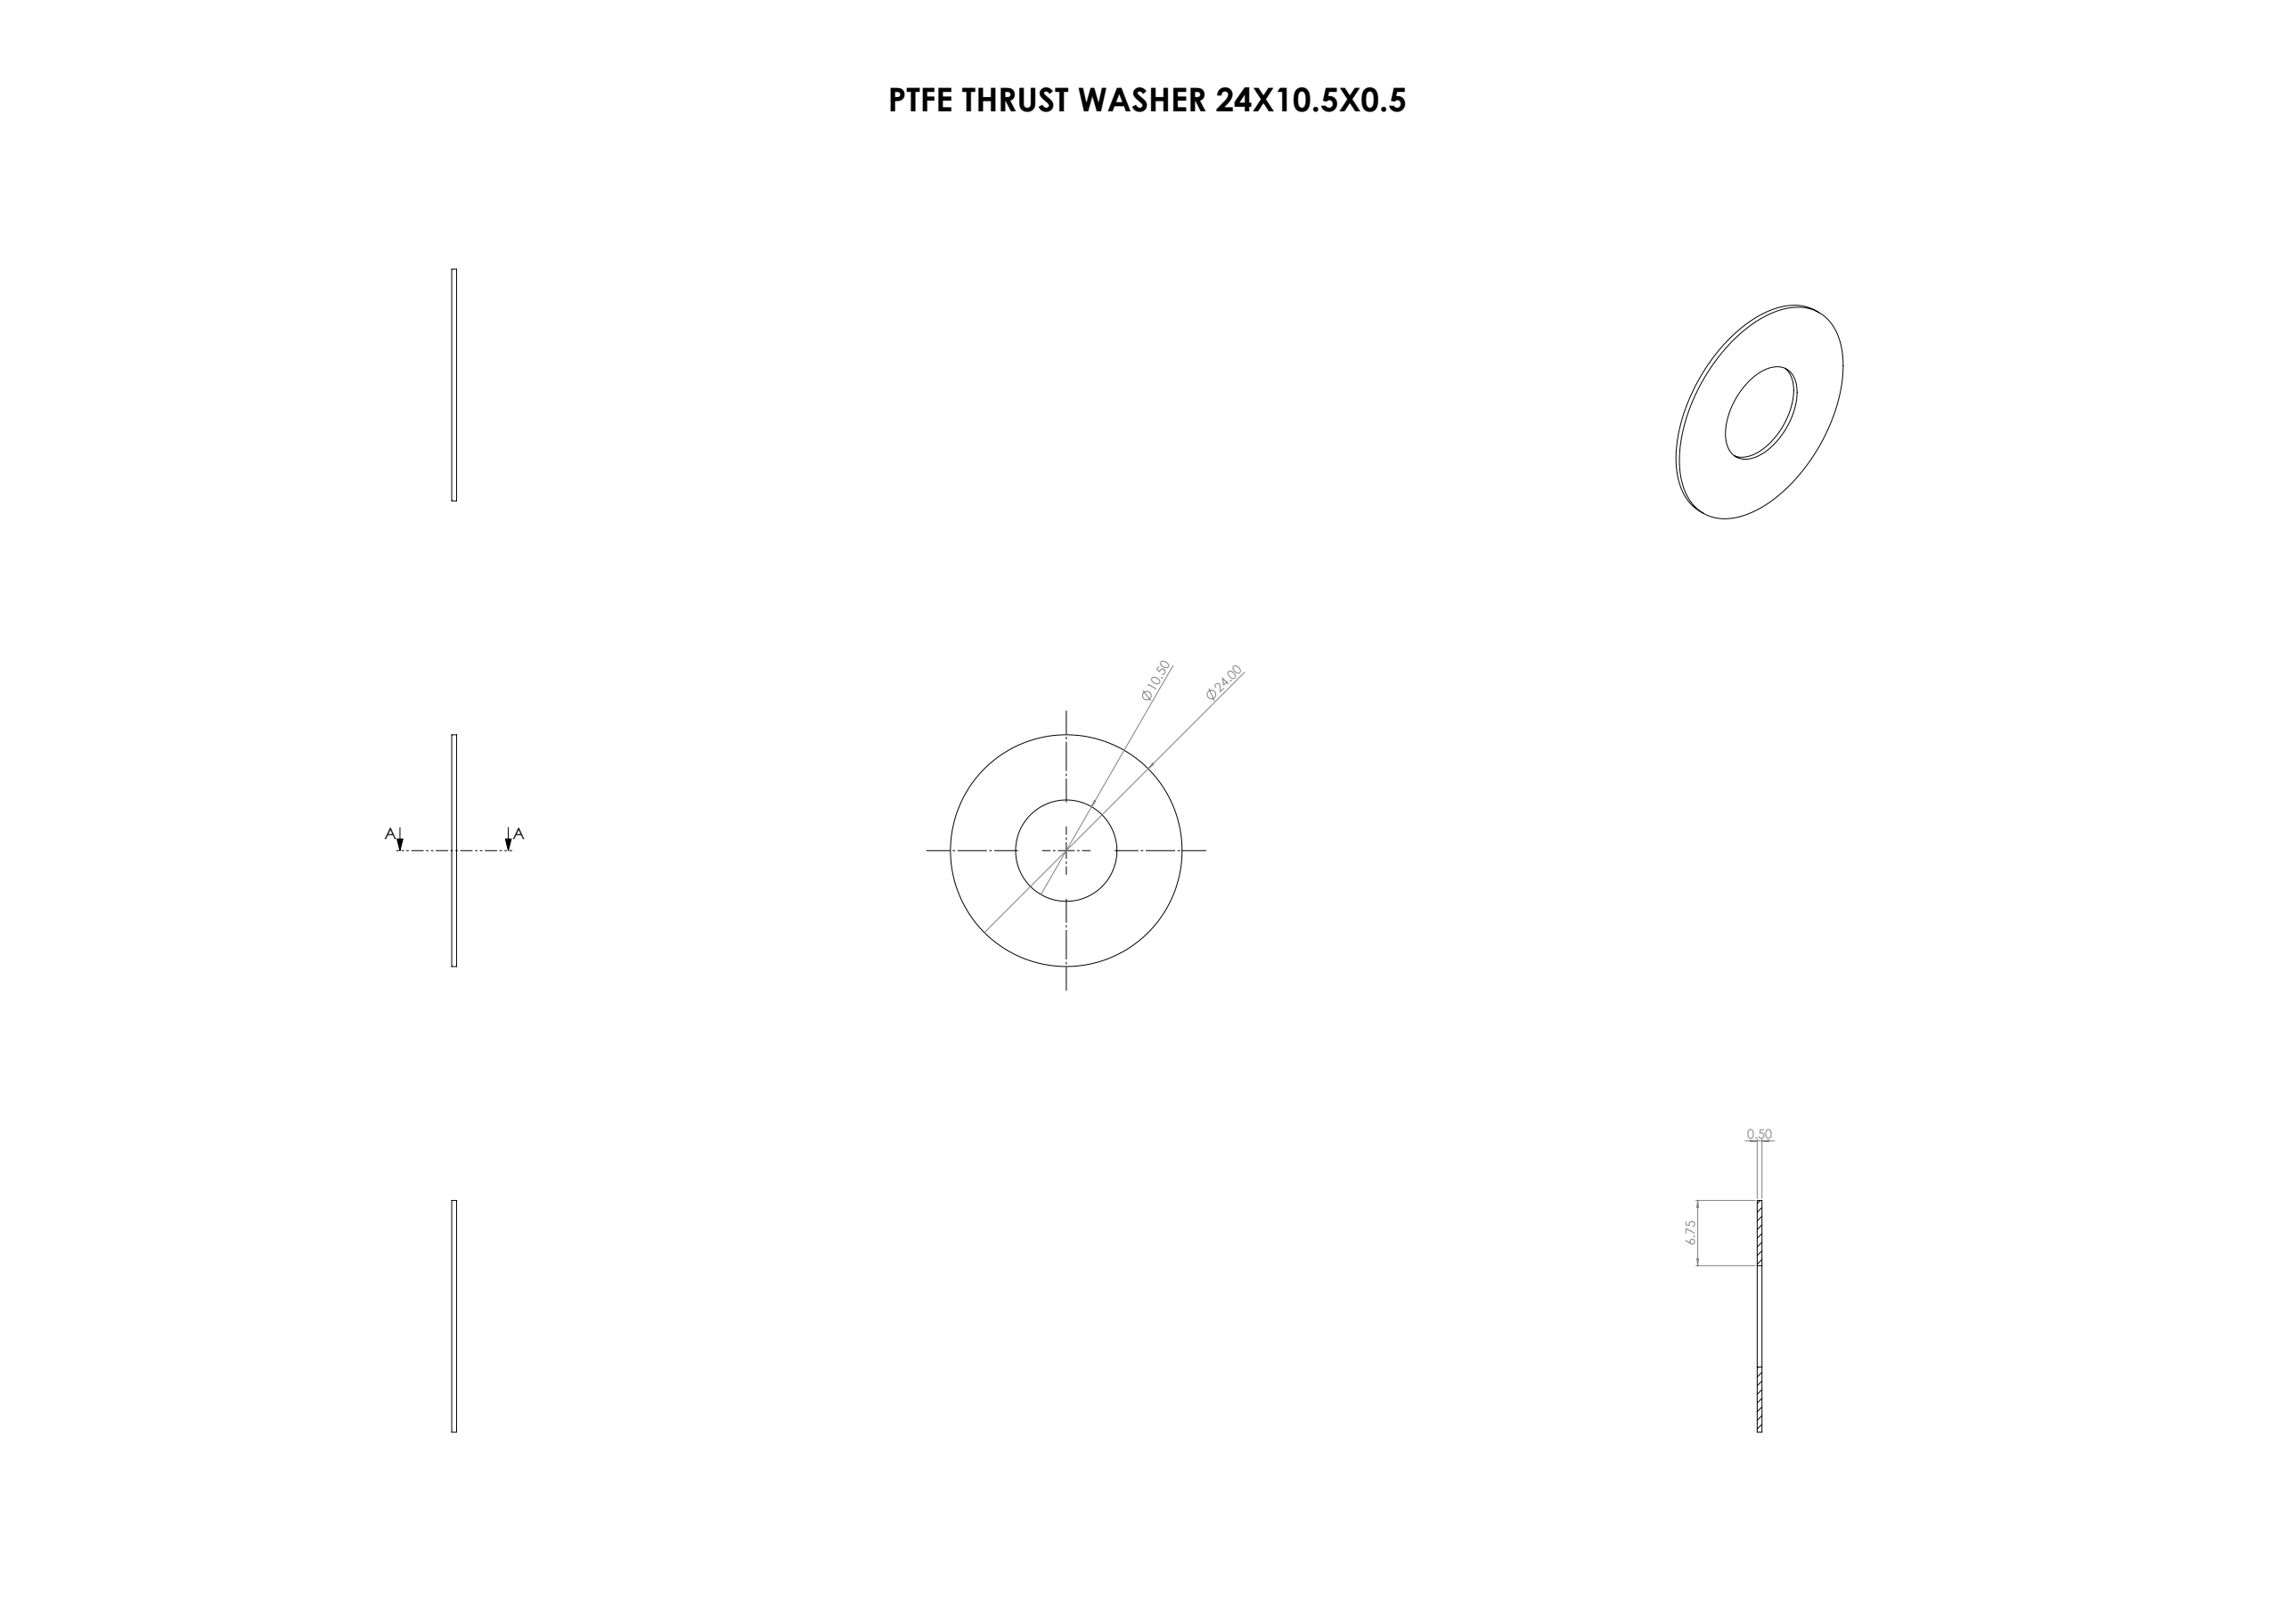
ISO-10303-21;
HEADER;
/* Generated by software containing ST-Developer
 * from STEP Tools, Inc. (www.steptools.com) 
 */

FILE_DESCRIPTION(
/* description */ (''),
/* implementation_level */ '2;1');

FILE_NAME(
/* name */ '06_PTFE_Thrust_Washer_24x10.5x0.5.step',
/* time_stamp */ '2026-10-21T02:03:06-07:00',
/* author */ (''),
/* organization */ (''),
/* preprocessor_version */ 'ST-DEVELOPER v20.2',
/* originating_system */ 'Autodesk Translation Framework v15.15.0.0',
/* authorisation */ '');

FILE_SCHEMA (('AUTOMOTIVE_DESIGN { 1 0 10303 214 3 1 1 }'));
ENDSEC;

DATA;
#10=MECHANICAL_DESIGN_GEOMETRIC_PRESENTATION_REPRESENTATION('',(#120),#38528);
#96=SHAPE_REPRESENTATION_RELATIONSHIP('SRR','None',#38581,#108);
#108=ADVANCED_BREP_SHAPE_REPRESENTATION('',(#132),#38521);
#120=STYLED_ITEM('',(#38713),#132);
#132=MANIFOLD_SOLID_BREP('Body1',#17077);
#381=CYLINDRICAL_SURFACE('',#18700,5.25);
#382=CYLINDRICAL_SURFACE('',#18705,12.);
#1469=FACE_BOUND('',#4078,.T.);
#1470=FACE_BOUND('',#4081,.T.);
#2173=CIRCLE('',#18701,5.25);
#2174=CIRCLE('',#18702,5.25);
#2175=CIRCLE('',#18704,12.);
#2176=CIRCLE('',#18706,12.);
#3056=FACE_OUTER_BOUND('',#4076,.T.);
#3057=FACE_OUTER_BOUND('',#4077,.T.);
#3058=FACE_OUTER_BOUND('',#4079,.T.);
#3059=FACE_OUTER_BOUND('',#4080,.T.);
#4076=EDGE_LOOP('',(#14519,#14520,#14521,#14522));
#4077=EDGE_LOOP('',(#14523));
#4078=EDGE_LOOP('',(#14524));
#4079=EDGE_LOOP('',(#14525,#14526,#14527,#14528));
#4080=EDGE_LOOP('',(#14529));
#4081=EDGE_LOOP('',(#14530));
#5026=LINE('',#33170,#6001);
#5027=LINE('',#33178,#6002);
#6001=VECTOR('',#22730,5.25);
#6002=VECTOR('',#22741,12.);
#7524=VERTEX_POINT('',#33167);
#7525=VERTEX_POINT('',#33169);
#7526=VERTEX_POINT('',#33173);
#7527=VERTEX_POINT('',#33176);
#9911=EDGE_CURVE('',#7524,#7524,#2173,.T.);
#9912=EDGE_CURVE('',#7524,#7525,#5026,.T.);
#9913=EDGE_CURVE('',#7525,#7525,#2174,.T.);
#9914=EDGE_CURVE('',#7526,#7526,#2175,.T.);
#9915=EDGE_CURVE('',#7527,#7527,#2176,.T.);
#9916=EDGE_CURVE('',#7527,#7526,#5027,.T.);
#14519=ORIENTED_EDGE('',*,*,#9911,.T.);
#14520=ORIENTED_EDGE('',*,*,#9912,.T.);
#14521=ORIENTED_EDGE('',*,*,#9913,.F.);
#14522=ORIENTED_EDGE('',*,*,#9912,.F.);
#14523=ORIENTED_EDGE('',*,*,#9914,.F.);
#14524=ORIENTED_EDGE('',*,*,#9913,.T.);
#14525=ORIENTED_EDGE('',*,*,#9915,.F.);
#14526=ORIENTED_EDGE('',*,*,#9916,.T.);
#14527=ORIENTED_EDGE('',*,*,#9914,.T.);
#14528=ORIENTED_EDGE('',*,*,#9916,.F.);
#14529=ORIENTED_EDGE('',*,*,#9915,.T.);
#14530=ORIENTED_EDGE('',*,*,#9911,.F.);
#15958=PLANE('',#18703);
#15959=PLANE('',#18707);
#16865=ADVANCED_FACE('',(#3056),#381,.F.);
#16866=ADVANCED_FACE('',(#3057,#1469),#15958,.T.);
#16867=ADVANCED_FACE('',(#3058),#382,.T.);
#16868=ADVANCED_FACE('',(#3059,#1470),#15959,.T.);
#17077=CLOSED_SHELL('',(#16865,#16866,#16867,#16868));
#18699=AXIS2_PLACEMENT_3D('',#33165,#22724,#22725);
#18700=AXIS2_PLACEMENT_3D('',#33166,#22726,#22727);
#18701=AXIS2_PLACEMENT_3D('',#33168,#22728,#22729);
#18702=AXIS2_PLACEMENT_3D('',#33171,#22731,#22732);
#18703=AXIS2_PLACEMENT_3D('',#33172,#22733,#22734);
#18704=AXIS2_PLACEMENT_3D('',#33174,#22735,#22736);
#18705=AXIS2_PLACEMENT_3D('',#33175,#22737,#22738);
#18706=AXIS2_PLACEMENT_3D('',#33177,#22739,#22740);
#18707=AXIS2_PLACEMENT_3D('',#33179,#22742,#22743);
#22724=DIRECTION('axis',(0.,0.,1.));
#22725=DIRECTION('refdir',(1.,0.,0.));
#22726=DIRECTION('center_axis',(1.,0.,0.));
#22727=DIRECTION('ref_axis',(0.,1.,0.));
#22728=DIRECTION('center_axis',(1.,0.,0.));
#22729=DIRECTION('ref_axis',(0.,0.,-1.));
#22730=DIRECTION('',(-1.,0.,0.));
#22731=DIRECTION('center_axis',(1.,0.,0.));
#22732=DIRECTION('ref_axis',(0.,0.,-1.));
#22733=DIRECTION('center_axis',(-1.,0.,0.));
#22734=DIRECTION('ref_axis',(0.,0.,1.));
#22735=DIRECTION('center_axis',(1.,0.,0.));
#22736=DIRECTION('ref_axis',(0.,0.,-1.));
#22737=DIRECTION('center_axis',(1.,0.,0.));
#22738=DIRECTION('ref_axis',(0.,1.,0.));
#22739=DIRECTION('center_axis',(1.,0.,0.));
#22740=DIRECTION('ref_axis',(0.,0.,-1.));
#22741=DIRECTION('',(-1.,0.,0.));
#22742=DIRECTION('center_axis',(1.,0.,0.));
#22743=DIRECTION('ref_axis',(0.,0.,-1.));
#33165=CARTESIAN_POINT('',(0.,0.,0.));
#33166=CARTESIAN_POINT('Origin',(0.25,0.,0.));
#33167=CARTESIAN_POINT('',(0.5,-5.25,-6.42939569552361E-16));
#33168=CARTESIAN_POINT('Origin',(0.5,0.,0.));
#33169=CARTESIAN_POINT('',(0.,-5.25,-6.42939569552361E-16));
#33170=CARTESIAN_POINT('',(0.25,-5.25,-6.42939569552361E-16));
#33171=CARTESIAN_POINT('Origin',(0.,0.,0.));
#33172=CARTESIAN_POINT('Origin',(0.,12.,0.));
#33173=CARTESIAN_POINT('',(0.,-12.,-1.46957615897682E-15));
#33174=CARTESIAN_POINT('Origin',(0.,0.,0.));
#33175=CARTESIAN_POINT('Origin',(0.25,0.,0.));
#33176=CARTESIAN_POINT('',(0.5,-12.,-1.46957615897682E-15));
#33177=CARTESIAN_POINT('Origin',(0.5,0.,0.));
#33178=CARTESIAN_POINT('',(0.25,-12.,-1.46957615897682E-15));
#33179=CARTESIAN_POINT('Origin',(0.5,5.25,0.));
#38507=UNCERTAINTY_MEASURE_WITH_UNIT(LENGTH_MEASURE(0.01),#38529,
'DISTANCE_ACCURACY_VALUE',
'Maximum model space distance between geometric entities at asserted c
onnectivities');
#38514=UNCERTAINTY_MEASURE_WITH_UNIT(LENGTH_MEASURE(0.01),#38529,
'DISTANCE_ACCURACY_VALUE',
'Maximum model space distance between geometric entities at asserted c
onnectivities');
#38521=(
GEOMETRIC_REPRESENTATION_CONTEXT(3)
GLOBAL_UNCERTAINTY_ASSIGNED_CONTEXT((#38507))
GLOBAL_UNIT_ASSIGNED_CONTEXT((#38529,#38531,#38532))
REPRESENTATION_CONTEXT('','3D')
);
#38528=(
GEOMETRIC_REPRESENTATION_CONTEXT(3)
GLOBAL_UNCERTAINTY_ASSIGNED_CONTEXT((#38514))
GLOBAL_UNIT_ASSIGNED_CONTEXT((#38529,#38531,#38532))
REPRESENTATION_CONTEXT('','3D')
);
#38529=(
LENGTH_UNIT()
NAMED_UNIT(*)
SI_UNIT(.MILLI.,.METRE.)
);
#38531=(
NAMED_UNIT(*)
PLANE_ANGLE_UNIT()
SI_UNIT($,.RADIAN.)
);
#38532=(
NAMED_UNIT(*)
SI_UNIT($,.STERADIAN.)
SOLID_ANGLE_UNIT()
);
#38539=SHAPE_DEFINITION_REPRESENTATION(#38552,#38581);
#38552=PRODUCT_DEFINITION_SHAPE('',$,#38595);
#38581=SHAPE_REPRESENTATION('',(#18699),#38521);
#38588=PRODUCT_DEFINITION_CONTEXT('part definition',#38629,'design');
#38595=PRODUCT_DEFINITION('2026-10-20-13-39-09-036',
'06_PTFE_Thrust_Washer_24x10.5x0.5',#38608,#38588);
#38608=PRODUCT_DEFINITION_FORMATION('',$,#38637);
#38629=APPLICATION_CONTEXT(
'Core Data for Automotive Mechanical Design Process');
#38630=PRODUCT_CONTEXT('part definition',#38629,'mechanical');
#38637=PRODUCT('2026-10-20-13-39-09-036',
'06_PTFE_Thrust_Washer_24x10.5x0.5',$,(#38630));
#38707=COLOUR_RGB('Black',0.12,0.14,0.17);
#38708=FILL_AREA_STYLE_COLOUR('',#38707);
#38709=FILL_AREA_STYLE('',(#38708));
#38710=SURFACE_STYLE_FILL_AREA(#38709);
#38711=SURFACE_SIDE_STYLE('',(#38710));
#38712=SURFACE_STYLE_USAGE(.BOTH.,#38711);
#38713=PRESENTATION_STYLE_ASSIGNMENT((#38712));
ENDSEC;
END-ISO-10303-21;
